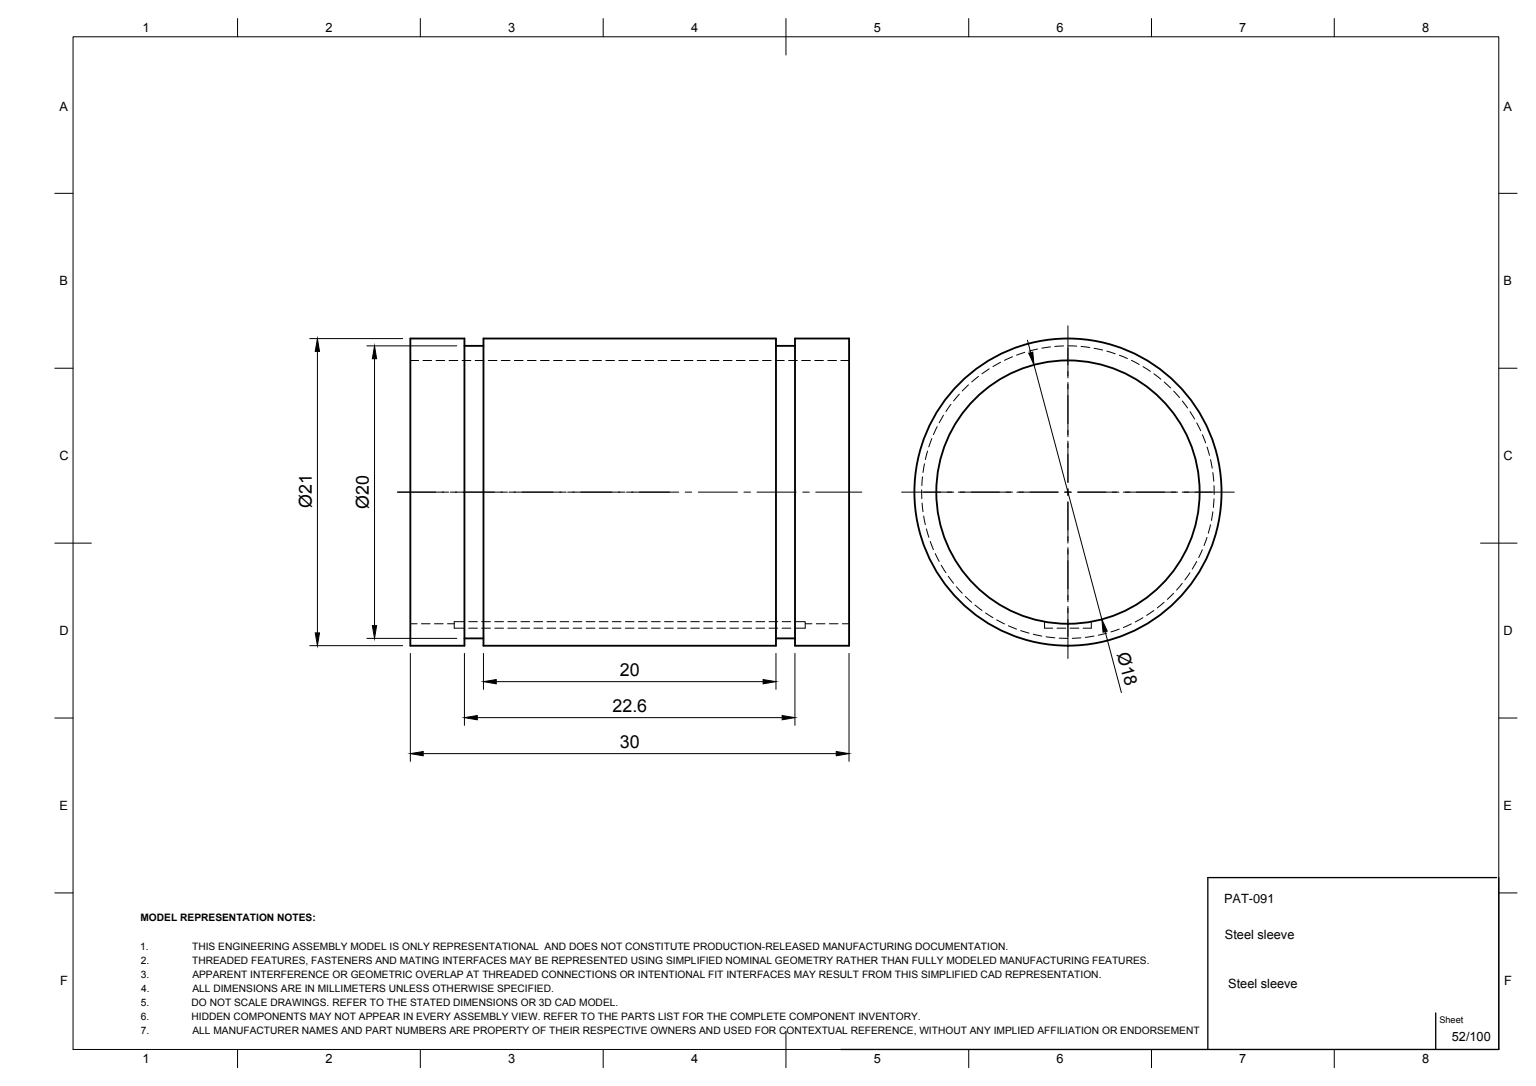
ISO-10303-21;
HEADER;
/* Generated by software containing ST-Developer
 * from STEP Tools, Inc. (www.steptools.com) 
 */

FILE_DESCRIPTION(
/* description */ ('PAT-091'),
/* implementation_level */ '2;1');

FILE_NAME(
/* name */ 'Steel sleeve.step',
/* time_stamp */ '2026-10-27T15:34:44-07:00',
/* author */ (''),
/* organization */ (''),
/* preprocessor_version */ 'ST-DEVELOPER v20.2',
/* originating_system */ 'Autodesk Translation Framework v15.17.0.0',
/* authorisation */ '');

FILE_SCHEMA (('AUTOMOTIVE_DESIGN { 1 0 10303 214 3 1 1 }'));
ENDSEC;

DATA;
#10=MECHANICAL_DESIGN_GEOMETRIC_PRESENTATION_REPRESENTATION('',(#1024),#25100);
#804=SHAPE_REPRESENTATION_RELATIONSHIP('SRR','None',#25569,#914);
#914=ADVANCED_BREP_SHAPE_REPRESENTATION('',(#1146),#25039);
#1024=STYLED_ITEM('',(#26205),#1146);
#1146=MANIFOLD_SOLID_BREP('Body1',#13303);
#1472=FACE_BOUND('',#3556,.T.);
#1473=FACE_BOUND('',#3559,.T.);
#1474=FACE_BOUND('',#3562,.T.);
#1475=FACE_BOUND('',#3565,.T.);
#1476=FACE_BOUND('',#3568,.T.);
#1477=FACE_BOUND('',#3571,.T.);
#1478=FACE_BOUND('',#3573,.T.);
#1869=PLANE('',#15420);
#1870=PLANE('',#15422);
#1871=PLANE('',#15423);
#1872=PLANE('',#15425);
#1873=PLANE('',#15426);
#1874=PLANE('',#15427);
#1875=PLANE('',#15432);
#1876=PLANE('',#15436);
#1877=PLANE('',#15440);
#1878=PLANE('',#15444);
#1879=PLANE('',#15448);
#2475=FACE_OUTER_BOUND('',#3550,.T.);
#2476=FACE_OUTER_BOUND('',#3551,.T.);
#2477=FACE_OUTER_BOUND('',#3552,.T.);
#2478=FACE_OUTER_BOUND('',#3553,.T.);
#2479=FACE_OUTER_BOUND('',#3554,.T.);
#2480=FACE_OUTER_BOUND('',#3555,.T.);
#2481=FACE_OUTER_BOUND('',#3557,.T.);
#2482=FACE_OUTER_BOUND('',#3558,.T.);
#2483=FACE_OUTER_BOUND('',#3560,.T.);
#2484=FACE_OUTER_BOUND('',#3561,.T.);
#2485=FACE_OUTER_BOUND('',#3563,.T.);
#2486=FACE_OUTER_BOUND('',#3564,.T.);
#2487=FACE_OUTER_BOUND('',#3566,.T.);
#2488=FACE_OUTER_BOUND('',#3567,.T.);
#2489=FACE_OUTER_BOUND('',#3569,.T.);
#2490=FACE_OUTER_BOUND('',#3570,.T.);
#2491=FACE_OUTER_BOUND('',#3572,.T.);
#3550=EDGE_LOOP('',(#10632,#10633,#10634,#10635));
#3551=EDGE_LOOP('',(#10636,#10637,#10638,#10639));
#3552=EDGE_LOOP('',(#10640,#10641,#10642,#10643));
#3553=EDGE_LOOP('',(#10644,#10645,#10646,#10647));
#3554=EDGE_LOOP('',(#10648,#10649,#10650,#10651));
#3555=EDGE_LOOP('',(#10652));
#3556=EDGE_LOOP('',(#10653));
#3557=EDGE_LOOP('',(#10654,#10655,#10656,#10657));
#3558=EDGE_LOOP('',(#10658));
#3559=EDGE_LOOP('',(#10659));
#3560=EDGE_LOOP('',(#10660,#10661,#10662,#10663));
#3561=EDGE_LOOP('',(#10664));
#3562=EDGE_LOOP('',(#10665));
#3563=EDGE_LOOP('',(#10666,#10667,#10668,#10669));
#3564=EDGE_LOOP('',(#10670));
#3565=EDGE_LOOP('',(#10671));
#3566=EDGE_LOOP('',(#10672,#10673,#10674,#10675));
#3567=EDGE_LOOP('',(#10676));
#3568=EDGE_LOOP('',(#10677));
#3569=EDGE_LOOP('',(#10678,#10679,#10680,#10681));
#3570=EDGE_LOOP('',(#10682));
#3571=EDGE_LOOP('',(#10683));
#3572=EDGE_LOOP('',(#10684,#10685,#10686,#10687));
#3573=EDGE_LOOP('',(#10688,#10689,#10690,#10691));
#4587=LINE('',#22884,#5327);
#4588=LINE('',#22886,#5328);
#4589=LINE('',#22887,#5329);
#4590=LINE('',#22890,#5330);
#4591=LINE('',#22892,#5331);
#4592=LINE('',#22893,#5332);
#4593=LINE('',#22898,#5333);
#4594=LINE('',#22899,#5334);
#4595=LINE('',#22901,#5335);
#4596=LINE('',#22902,#5336);
#4597=LINE('',#22912,#5337);
#4598=LINE('',#22919,#5338);
#4599=LINE('',#22926,#5339);
#4600=LINE('',#22933,#5340);
#4601=LINE('',#22940,#5341);
#4602=LINE('',#22945,#5342);
#5327=VECTOR('',#18605,1.);
#5328=VECTOR('',#18606,1.);
#5329=VECTOR('',#18607,1.);
#5330=VECTOR('',#18610,1.);
#5331=VECTOR('',#18611,1.);
#5332=VECTOR('',#18612,1.);
#5333=VECTOR('',#18617,1.);
#5334=VECTOR('',#18618,1.);
#5335=VECTOR('',#18621,1.);
#5336=VECTOR('',#18622,1.);
#5337=VECTOR('',#18635,1.05);
#5338=VECTOR('',#18644,1.);
#5339=VECTOR('',#18653,1.05);
#5340=VECTOR('',#18662,1.);
#5341=VECTOR('',#18671,1.05);
#5342=VECTOR('',#18678,0.9);
#5967=CIRCLE('',#15421,0.9);
#5968=CIRCLE('',#15424,0.9);
#5969=CIRCLE('',#15428,1.05);
#5970=CIRCLE('',#15429,0.9);
#5971=CIRCLE('',#15431,1.05);
#5972=CIRCLE('',#15433,1.);
#5973=CIRCLE('',#15435,1.);
#5974=CIRCLE('',#15437,1.05);
#5975=CIRCLE('',#15439,1.05);
#5976=CIRCLE('',#15441,1.);
#5977=CIRCLE('',#15443,1.);
#5978=CIRCLE('',#15445,1.05);
#5979=CIRCLE('',#15447,1.05);
#5980=CIRCLE('',#15449,0.9);
#6934=VERTEX_POINT('',#22880);
#6935=VERTEX_POINT('',#22881);
#6936=VERTEX_POINT('',#22883);
#6937=VERTEX_POINT('',#22885);
#6938=VERTEX_POINT('',#22889);
#6939=VERTEX_POINT('',#22891);
#6940=VERTEX_POINT('',#22895);
#6941=VERTEX_POINT('',#22897);
#6942=VERTEX_POINT('',#22905);
#6943=VERTEX_POINT('',#22907);
#6944=VERTEX_POINT('',#22910);
#6945=VERTEX_POINT('',#22914);
#6946=VERTEX_POINT('',#22917);
#6947=VERTEX_POINT('',#22921);
#6948=VERTEX_POINT('',#22924);
#6949=VERTEX_POINT('',#22928);
#6950=VERTEX_POINT('',#22931);
#6951=VERTEX_POINT('',#22935);
#6952=VERTEX_POINT('',#22938);
#6953=VERTEX_POINT('',#22942);
#8251=EDGE_CURVE('',#6934,#6935,#5967,.T.);
#8252=EDGE_CURVE('',#6936,#6934,#4587,.T.);
#8253=EDGE_CURVE('',#6937,#6936,#4588,.T.);
#8254=EDGE_CURVE('',#6935,#6937,#4589,.T.);
#8255=EDGE_CURVE('',#6935,#6938,#4590,.T.);
#8256=EDGE_CURVE('',#6939,#6937,#4591,.T.);
#8257=EDGE_CURVE('',#6939,#6938,#4592,.T.);
#8258=EDGE_CURVE('',#6938,#6940,#5968,.T.);
#8259=EDGE_CURVE('',#6941,#6939,#4593,.T.);
#8260=EDGE_CURVE('',#6940,#6941,#4594,.T.);
#8261=EDGE_CURVE('',#6940,#6934,#4595,.T.);
#8262=EDGE_CURVE('',#6941,#6936,#4596,.T.);
#8263=EDGE_CURVE('',#6942,#6942,#5969,.T.);
#8264=EDGE_CURVE('',#6943,#6943,#5970,.T.);
#8265=EDGE_CURVE('',#6944,#6944,#5971,.T.);
#8266=EDGE_CURVE('',#6944,#6942,#4597,.T.);
#8267=EDGE_CURVE('',#6945,#6945,#5972,.T.);
#8268=EDGE_CURVE('',#6946,#6946,#5973,.T.);
#8269=EDGE_CURVE('',#6946,#6945,#4598,.T.);
#8270=EDGE_CURVE('',#6947,#6947,#5974,.T.);
#8271=EDGE_CURVE('',#6948,#6948,#5975,.T.);
#8272=EDGE_CURVE('',#6948,#6947,#4599,.T.);
#8273=EDGE_CURVE('',#6949,#6949,#5976,.T.);
#8274=EDGE_CURVE('',#6950,#6950,#5977,.T.);
#8275=EDGE_CURVE('',#6950,#6949,#4600,.T.);
#8276=EDGE_CURVE('',#6951,#6951,#5978,.T.);
#8277=EDGE_CURVE('',#6952,#6952,#5979,.T.);
#8278=EDGE_CURVE('',#6952,#6951,#4601,.T.);
#8279=EDGE_CURVE('',#6953,#6953,#5980,.T.);
#8280=EDGE_CURVE('',#6953,#6943,#4602,.T.);
#10632=ORIENTED_EDGE('',*,*,#8251,.F.);
#10633=ORIENTED_EDGE('',*,*,#8252,.F.);
#10634=ORIENTED_EDGE('',*,*,#8253,.F.);
#10635=ORIENTED_EDGE('',*,*,#8254,.F.);
#10636=ORIENTED_EDGE('',*,*,#8255,.F.);
#10637=ORIENTED_EDGE('',*,*,#8254,.T.);
#10638=ORIENTED_EDGE('',*,*,#8256,.F.);
#10639=ORIENTED_EDGE('',*,*,#8257,.T.);
#10640=ORIENTED_EDGE('',*,*,#8258,.F.);
#10641=ORIENTED_EDGE('',*,*,#8257,.F.);
#10642=ORIENTED_EDGE('',*,*,#8259,.F.);
#10643=ORIENTED_EDGE('',*,*,#8260,.F.);
#10644=ORIENTED_EDGE('',*,*,#8261,.F.);
#10645=ORIENTED_EDGE('',*,*,#8260,.T.);
#10646=ORIENTED_EDGE('',*,*,#8262,.T.);
#10647=ORIENTED_EDGE('',*,*,#8252,.T.);
#10648=ORIENTED_EDGE('',*,*,#8262,.F.);
#10649=ORIENTED_EDGE('',*,*,#8259,.T.);
#10650=ORIENTED_EDGE('',*,*,#8256,.T.);
#10651=ORIENTED_EDGE('',*,*,#8253,.T.);
#10652=ORIENTED_EDGE('',*,*,#8263,.F.);
#10653=ORIENTED_EDGE('',*,*,#8264,.T.);
#10654=ORIENTED_EDGE('',*,*,#8265,.F.);
#10655=ORIENTED_EDGE('',*,*,#8266,.T.);
#10656=ORIENTED_EDGE('',*,*,#8263,.T.);
#10657=ORIENTED_EDGE('',*,*,#8266,.F.);
#10658=ORIENTED_EDGE('',*,*,#8265,.T.);
#10659=ORIENTED_EDGE('',*,*,#8267,.F.);
#10660=ORIENTED_EDGE('',*,*,#8268,.F.);
#10661=ORIENTED_EDGE('',*,*,#8269,.T.);
#10662=ORIENTED_EDGE('',*,*,#8267,.T.);
#10663=ORIENTED_EDGE('',*,*,#8269,.F.);
#10664=ORIENTED_EDGE('',*,*,#8270,.F.);
#10665=ORIENTED_EDGE('',*,*,#8268,.T.);
#10666=ORIENTED_EDGE('',*,*,#8271,.F.);
#10667=ORIENTED_EDGE('',*,*,#8272,.T.);
#10668=ORIENTED_EDGE('',*,*,#8270,.T.);
#10669=ORIENTED_EDGE('',*,*,#8272,.F.);
#10670=ORIENTED_EDGE('',*,*,#8271,.T.);
#10671=ORIENTED_EDGE('',*,*,#8273,.F.);
#10672=ORIENTED_EDGE('',*,*,#8274,.F.);
#10673=ORIENTED_EDGE('',*,*,#8275,.T.);
#10674=ORIENTED_EDGE('',*,*,#8273,.T.);
#10675=ORIENTED_EDGE('',*,*,#8275,.F.);
#10676=ORIENTED_EDGE('',*,*,#8276,.F.);
#10677=ORIENTED_EDGE('',*,*,#8274,.T.);
#10678=ORIENTED_EDGE('',*,*,#8277,.F.);
#10679=ORIENTED_EDGE('',*,*,#8278,.T.);
#10680=ORIENTED_EDGE('',*,*,#8276,.T.);
#10681=ORIENTED_EDGE('',*,*,#8278,.F.);
#10682=ORIENTED_EDGE('',*,*,#8277,.T.);
#10683=ORIENTED_EDGE('',*,*,#8279,.F.);
#10684=ORIENTED_EDGE('',*,*,#8279,.T.);
#10685=ORIENTED_EDGE('',*,*,#8280,.T.);
#10686=ORIENTED_EDGE('',*,*,#8264,.F.);
#10687=ORIENTED_EDGE('',*,*,#8280,.F.);
#10688=ORIENTED_EDGE('',*,*,#8258,.T.);
#10689=ORIENTED_EDGE('',*,*,#8261,.T.);
#10690=ORIENTED_EDGE('',*,*,#8251,.T.);
#10691=ORIENTED_EDGE('',*,*,#8255,.T.);
#12250=CYLINDRICAL_SURFACE('',#15430,1.05);
#12251=CYLINDRICAL_SURFACE('',#15434,1.);
#12252=CYLINDRICAL_SURFACE('',#15438,1.05);
#12253=CYLINDRICAL_SURFACE('',#15442,1.);
#12254=CYLINDRICAL_SURFACE('',#15446,1.05);
#12255=CYLINDRICAL_SURFACE('',#15450,0.9);
#12842=ADVANCED_FACE('',(#2475),#1869,.F.);
#12843=ADVANCED_FACE('',(#2476),#1870,.F.);
#12844=ADVANCED_FACE('',(#2477),#1871,.F.);
#12845=ADVANCED_FACE('',(#2478),#1872,.F.);
#12846=ADVANCED_FACE('',(#2479),#1873,.F.);
#12847=ADVANCED_FACE('',(#2480,#1472),#1874,.T.);
#12848=ADVANCED_FACE('',(#2481),#12250,.T.);
#12849=ADVANCED_FACE('',(#2482,#1473),#1875,.T.);
#12850=ADVANCED_FACE('',(#2483),#12251,.T.);
#12851=ADVANCED_FACE('',(#2484,#1474),#1876,.T.);
#12852=ADVANCED_FACE('',(#2485),#12252,.T.);
#12853=ADVANCED_FACE('',(#2486,#1475),#1877,.T.);
#12854=ADVANCED_FACE('',(#2487),#12253,.T.);
#12855=ADVANCED_FACE('',(#2488,#1476),#1878,.T.);
#12856=ADVANCED_FACE('',(#2489),#12254,.T.);
#12857=ADVANCED_FACE('',(#2490,#1477),#1879,.T.);
#12858=ADVANCED_FACE('',(#2491,#1478),#12255,.F.);
#13303=CLOSED_SHELL('',(#12842,#12843,#12844,#12845,#12846,#12847,#12848,
#12849,#12850,#12851,#12852,#12853,#12854,#12855,#12856,#12857,#12858));
#15419=AXIS2_PLACEMENT_3D('',#22878,#18599,#18600);
#15420=AXIS2_PLACEMENT_3D('',#22879,#18601,#18602);
#15421=AXIS2_PLACEMENT_3D('',#22882,#18603,#18604);
#15422=AXIS2_PLACEMENT_3D('',#22888,#18608,#18609);
#15423=AXIS2_PLACEMENT_3D('',#22894,#18613,#18614);
#15424=AXIS2_PLACEMENT_3D('',#22896,#18615,#18616);
#15425=AXIS2_PLACEMENT_3D('',#22900,#18619,#18620);
#15426=AXIS2_PLACEMENT_3D('',#22903,#18623,#18624);
#15427=AXIS2_PLACEMENT_3D('',#22904,#18625,#18626);
#15428=AXIS2_PLACEMENT_3D('',#22906,#18627,#18628);
#15429=AXIS2_PLACEMENT_3D('',#22908,#18629,#18630);
#15430=AXIS2_PLACEMENT_3D('',#22909,#18631,#18632);
#15431=AXIS2_PLACEMENT_3D('',#22911,#18633,#18634);
#15432=AXIS2_PLACEMENT_3D('',#22913,#18636,#18637);
#15433=AXIS2_PLACEMENT_3D('',#22915,#18638,#18639);
#15434=AXIS2_PLACEMENT_3D('',#22916,#18640,#18641);
#15435=AXIS2_PLACEMENT_3D('',#22918,#18642,#18643);
#15436=AXIS2_PLACEMENT_3D('',#22920,#18645,#18646);
#15437=AXIS2_PLACEMENT_3D('',#22922,#18647,#18648);
#15438=AXIS2_PLACEMENT_3D('',#22923,#18649,#18650);
#15439=AXIS2_PLACEMENT_3D('',#22925,#18651,#18652);
#15440=AXIS2_PLACEMENT_3D('',#22927,#18654,#18655);
#15441=AXIS2_PLACEMENT_3D('',#22929,#18656,#18657);
#15442=AXIS2_PLACEMENT_3D('',#22930,#18658,#18659);
#15443=AXIS2_PLACEMENT_3D('',#22932,#18660,#18661);
#15444=AXIS2_PLACEMENT_3D('',#22934,#18663,#18664);
#15445=AXIS2_PLACEMENT_3D('',#22936,#18665,#18666);
#15446=AXIS2_PLACEMENT_3D('',#22937,#18667,#18668);
#15447=AXIS2_PLACEMENT_3D('',#22939,#18669,#18670);
#15448=AXIS2_PLACEMENT_3D('',#22941,#18672,#18673);
#15449=AXIS2_PLACEMENT_3D('',#22943,#18674,#18675);
#15450=AXIS2_PLACEMENT_3D('',#22944,#18676,#18677);
#18599=DIRECTION('axis',(0.,0.,1.));
#18600=DIRECTION('refdir',(1.,0.,0.));
#18601=DIRECTION('center_axis',(0.,1.,0.));
#18602=DIRECTION('ref_axis',(0.,0.,1.));
#18603=DIRECTION('center_axis',(0.,-1.,0.));
#18604=DIRECTION('ref_axis',(1.,0.,0.));
#18605=DIRECTION('',(-1.,0.,0.));
#18606=DIRECTION('',(0.,0.,-1.));
#18607=DIRECTION('',(1.,0.,0.));
#18608=DIRECTION('center_axis',(0.,0.,1.));
#18609=DIRECTION('ref_axis',(1.,0.,0.));
#18610=DIRECTION('',(0.,-1.,0.));
#18611=DIRECTION('',(0.,1.,0.));
#18612=DIRECTION('',(-1.,0.,0.));
#18613=DIRECTION('center_axis',(0.,-1.,0.));
#18614=DIRECTION('ref_axis',(0.,0.,-1.));
#18615=DIRECTION('center_axis',(0.,1.,0.));
#18616=DIRECTION('ref_axis',(1.,0.,0.));
#18617=DIRECTION('',(0.,0.,1.));
#18618=DIRECTION('',(1.,0.,0.));
#18619=DIRECTION('center_axis',(0.,0.,-1.));
#18620=DIRECTION('ref_axis',(-1.,0.,0.));
#18621=DIRECTION('',(0.,1.,0.));
#18622=DIRECTION('',(0.,1.,0.));
#18623=DIRECTION('center_axis',(1.,0.,0.));
#18624=DIRECTION('ref_axis',(0.,0.,-1.));
#18625=DIRECTION('center_axis',(0.,1.,0.));
#18626=DIRECTION('ref_axis',(0.,0.,1.));
#18627=DIRECTION('center_axis',(0.,-1.,0.));
#18628=DIRECTION('ref_axis',(1.,0.,0.));
#18629=DIRECTION('center_axis',(0.,-1.,0.));
#18630=DIRECTION('ref_axis',(1.,0.,0.));
#18631=DIRECTION('center_axis',(0.,-1.,0.));
#18632=DIRECTION('ref_axis',(1.,0.,0.));
#18633=DIRECTION('center_axis',(0.,-1.,0.));
#18634=DIRECTION('ref_axis',(1.,0.,0.));
#18635=DIRECTION('',(0.,1.,0.));
#18636=DIRECTION('center_axis',(0.,-1.,0.));
#18637=DIRECTION('ref_axis',(0.,0.,-1.));
#18638=DIRECTION('center_axis',(0.,-1.,0.));
#18639=DIRECTION('ref_axis',(1.,0.,0.));
#18640=DIRECTION('center_axis',(0.,-1.,0.));
#18641=DIRECTION('ref_axis',(1.,0.,0.));
#18642=DIRECTION('center_axis',(0.,-1.,0.));
#18643=DIRECTION('ref_axis',(1.,0.,0.));
#18644=DIRECTION('',(0.,1.,0.));
#18645=DIRECTION('center_axis',(0.,1.,0.));
#18646=DIRECTION('ref_axis',(0.,0.,1.));
#18647=DIRECTION('center_axis',(0.,-1.,0.));
#18648=DIRECTION('ref_axis',(1.,0.,0.));
#18649=DIRECTION('center_axis',(0.,-1.,0.));
#18650=DIRECTION('ref_axis',(1.,0.,0.));
#18651=DIRECTION('center_axis',(0.,-1.,0.));
#18652=DIRECTION('ref_axis',(1.,0.,0.));
#18653=DIRECTION('',(0.,1.,0.));
#18654=DIRECTION('center_axis',(0.,-1.,0.));
#18655=DIRECTION('ref_axis',(0.,0.,-1.));
#18656=DIRECTION('center_axis',(0.,-1.,0.));
#18657=DIRECTION('ref_axis',(1.,0.,0.));
#18658=DIRECTION('center_axis',(0.,-1.,0.));
#18659=DIRECTION('ref_axis',(1.,0.,0.));
#18660=DIRECTION('center_axis',(0.,-1.,0.));
#18661=DIRECTION('ref_axis',(1.,0.,0.));
#18662=DIRECTION('',(0.,1.,0.));
#18663=DIRECTION('center_axis',(0.,1.,0.));
#18664=DIRECTION('ref_axis',(0.,0.,1.));
#18665=DIRECTION('center_axis',(0.,-1.,0.));
#18666=DIRECTION('ref_axis',(1.,0.,0.));
#18667=DIRECTION('center_axis',(0.,-1.,0.));
#18668=DIRECTION('ref_axis',(1.,0.,0.));
#18669=DIRECTION('center_axis',(0.,-1.,0.));
#18670=DIRECTION('ref_axis',(1.,0.,0.));
#18671=DIRECTION('',(0.,1.,0.));
#18672=DIRECTION('center_axis',(0.,-1.,0.));
#18673=DIRECTION('ref_axis',(0.,0.,-1.));
#18674=DIRECTION('center_axis',(0.,-1.,0.));
#18675=DIRECTION('ref_axis',(1.,0.,0.));
#18676=DIRECTION('center_axis',(0.,-1.,0.));
#18677=DIRECTION('ref_axis',(1.,0.,0.));
#18678=DIRECTION('',(0.,1.,0.));
#22878=CARTESIAN_POINT('',(0.,0.,0.));
#22879=CARTESIAN_POINT('Origin',(0.75,1.2,0.));
#22880=CARTESIAN_POINT('',(0.885663593019381,1.2,-0.16));
#22881=CARTESIAN_POINT('',(0.885663593019381,1.2,0.16));
#22882=CARTESIAN_POINT('Origin',(0.,1.2,0.));
#22883=CARTESIAN_POINT('',(0.93,1.2,-0.16));
#22884=CARTESIAN_POINT('',(0.93,1.2,-0.16));
#22885=CARTESIAN_POINT('',(0.93,1.2,0.16));
#22886=CARTESIAN_POINT('',(0.93,1.2,0.16));
#22887=CARTESIAN_POINT('',(0.57,1.2,0.16));
#22888=CARTESIAN_POINT('Origin',(0.57,0.,0.16));
#22889=CARTESIAN_POINT('',(0.885663593019381,-1.2,0.16));
#22890=CARTESIAN_POINT('',(0.885663593019381,0.,0.16));
#22891=CARTESIAN_POINT('',(0.93,-1.2,0.16));
#22892=CARTESIAN_POINT('',(0.93,0.,0.16));
#22893=CARTESIAN_POINT('',(0.57,-1.2,0.16));
#22894=CARTESIAN_POINT('Origin',(0.75,-1.2,0.));
#22895=CARTESIAN_POINT('',(0.885663593019381,-1.2,-0.16));
#22896=CARTESIAN_POINT('Origin',(0.,-1.2,0.));
#22897=CARTESIAN_POINT('',(0.93,-1.2,-0.16));
#22898=CARTESIAN_POINT('',(0.93,-1.2,0.16));
#22899=CARTESIAN_POINT('',(0.93,-1.2,-0.16));
#22900=CARTESIAN_POINT('Origin',(0.93,0.,-0.16));
#22901=CARTESIAN_POINT('',(0.885663593019381,0.,-0.16));
#22902=CARTESIAN_POINT('',(0.93,0.,-0.16));
#22903=CARTESIAN_POINT('Origin',(0.93,0.,0.16));
#22904=CARTESIAN_POINT('Origin',(1.05,1.5,0.));
#22905=CARTESIAN_POINT('',(-1.05,1.5,-1.28587913910472E-16));
#22906=CARTESIAN_POINT('Origin',(0.,1.5,0.));
#22907=CARTESIAN_POINT('',(-0.9,1.5,-1.10218211923262E-16));
#22908=CARTESIAN_POINT('Origin',(0.,1.5,0.));
#22909=CARTESIAN_POINT('Origin',(0.,1.315,0.));
#22910=CARTESIAN_POINT('',(-1.05,1.13,-1.28587913910472E-16));
#22911=CARTESIAN_POINT('Origin',(0.,1.13,0.));
#22912=CARTESIAN_POINT('',(-1.05,1.315,-1.28587913910472E-16));
#22913=CARTESIAN_POINT('Origin',(1.,1.13,0.));
#22914=CARTESIAN_POINT('',(-1.,1.13,-1.22464679914735E-16));
#22915=CARTESIAN_POINT('Origin',(0.,1.13,0.));
#22916=CARTESIAN_POINT('Origin',(0.,1.065,0.));
#22917=CARTESIAN_POINT('',(-1.,1.,-1.22464679914735E-16));
#22918=CARTESIAN_POINT('Origin',(0.,1.,0.));
#22919=CARTESIAN_POINT('',(-1.,1.065,-1.22464679914735E-16));
#22920=CARTESIAN_POINT('Origin',(1.05,1.,0.));
#22921=CARTESIAN_POINT('',(-1.05,1.,-1.28587913910472E-16));
#22922=CARTESIAN_POINT('Origin',(0.,1.,0.));
#22923=CARTESIAN_POINT('Origin',(0.,0.,0.));
#22924=CARTESIAN_POINT('',(-1.05,-1.,-1.28587913910472E-16));
#22925=CARTESIAN_POINT('Origin',(0.,-1.,0.));
#22926=CARTESIAN_POINT('',(-1.05,0.,-1.28587913910472E-16));
#22927=CARTESIAN_POINT('Origin',(1.,-1.,0.));
#22928=CARTESIAN_POINT('',(-1.,-1.,-1.22464679914735E-16));
#22929=CARTESIAN_POINT('Origin',(0.,-1.,0.));
#22930=CARTESIAN_POINT('Origin',(0.,-1.065,0.));
#22931=CARTESIAN_POINT('',(-1.,-1.13,-1.22464679914735E-16));
#22932=CARTESIAN_POINT('Origin',(0.,-1.13,0.));
#22933=CARTESIAN_POINT('',(-1.,-1.065,-1.22464679914735E-16));
#22934=CARTESIAN_POINT('Origin',(1.05,-1.13,0.));
#22935=CARTESIAN_POINT('',(-1.05,-1.13,-1.28587913910472E-16));
#22936=CARTESIAN_POINT('Origin',(0.,-1.13,0.));
#22937=CARTESIAN_POINT('Origin',(0.,-1.315,0.));
#22938=CARTESIAN_POINT('',(-1.05,-1.5,-1.28587913910472E-16));
#22939=CARTESIAN_POINT('Origin',(0.,-1.5,0.));
#22940=CARTESIAN_POINT('',(-1.05,-1.315,-1.28587913910472E-16));
#22941=CARTESIAN_POINT('Origin',(0.9,-1.5,0.));
#22942=CARTESIAN_POINT('',(-0.9,-1.5,-1.10218211923262E-16));
#22943=CARTESIAN_POINT('Origin',(0.,-1.5,0.));
#22944=CARTESIAN_POINT('Origin',(0.,0.,0.));
#22945=CARTESIAN_POINT('',(-0.9,0.,-1.10218211923262E-16));
#24918=UNCERTAINTY_MEASURE_WITH_UNIT(LENGTH_MEASURE(0.001),#25101,
'DISTANCE_ACCURACY_VALUE',
'Maximum model space distance between geometric entities at asserted c
onnectivities');
#24979=UNCERTAINTY_MEASURE_WITH_UNIT(LENGTH_MEASURE(0.001),#25101,
'DISTANCE_ACCURACY_VALUE',
'Maximum model space distance between geometric entities at asserted c
onnectivities');
#25039=(
GEOMETRIC_REPRESENTATION_CONTEXT(3)
GLOBAL_UNCERTAINTY_ASSIGNED_CONTEXT((#24918))
GLOBAL_UNIT_ASSIGNED_CONTEXT((#25101,#25103,#25104))
REPRESENTATION_CONTEXT('','3D')
);
#25100=(
GEOMETRIC_REPRESENTATION_CONTEXT(3)
GLOBAL_UNCERTAINTY_ASSIGNED_CONTEXT((#24979))
GLOBAL_UNIT_ASSIGNED_CONTEXT((#25101,#25103,#25104))
REPRESENTATION_CONTEXT('','3D')
);
#25101=(
LENGTH_UNIT()
NAMED_UNIT(*)
SI_UNIT(.CENTI.,.METRE.)
);
#25103=(
NAMED_UNIT(*)
PLANE_ANGLE_UNIT()
SI_UNIT($,.RADIAN.)
);
#25104=(
NAMED_UNIT(*)
SI_UNIT($,.STERADIAN.)
SOLID_ANGLE_UNIT()
);
#25164=SHAPE_DEFINITION_REPRESENTATION(#25284,#25569);
#25284=PRODUCT_DEFINITION_SHAPE('',$,#25690);
#25569=SHAPE_REPRESENTATION('',(#15419),#25039);
#25630=PRODUCT_DEFINITION_CONTEXT('part definition',#25992,'design');
#25690=PRODUCT_DEFINITION('Steel sleeve','Steel sleeve',#25810,#25630);
#25810=PRODUCT_DEFINITION_FORMATION('',$,#26053);
#25992=APPLICATION_CONTEXT(
'Core Data for Automotive Mechanical Design Process');
#25993=PRODUCT_CONTEXT('part definition',#25992,'mechanical');
#26053=PRODUCT('Steel sleeve','Steel sleeve','Steel sleeve',(#25993));
#26199=COLOUR_RGB('Off White',0.89,0.88,0.83);
#26200=FILL_AREA_STYLE_COLOUR('',#26199);
#26201=FILL_AREA_STYLE('',(#26200));
#26202=SURFACE_STYLE_FILL_AREA(#26201);
#26203=SURFACE_SIDE_STYLE('',(#26202));
#26204=SURFACE_STYLE_USAGE(.BOTH.,#26203);
#26205=PRESENTATION_STYLE_ASSIGNMENT((#26204));
ENDSEC;
END-ISO-10303-21;
